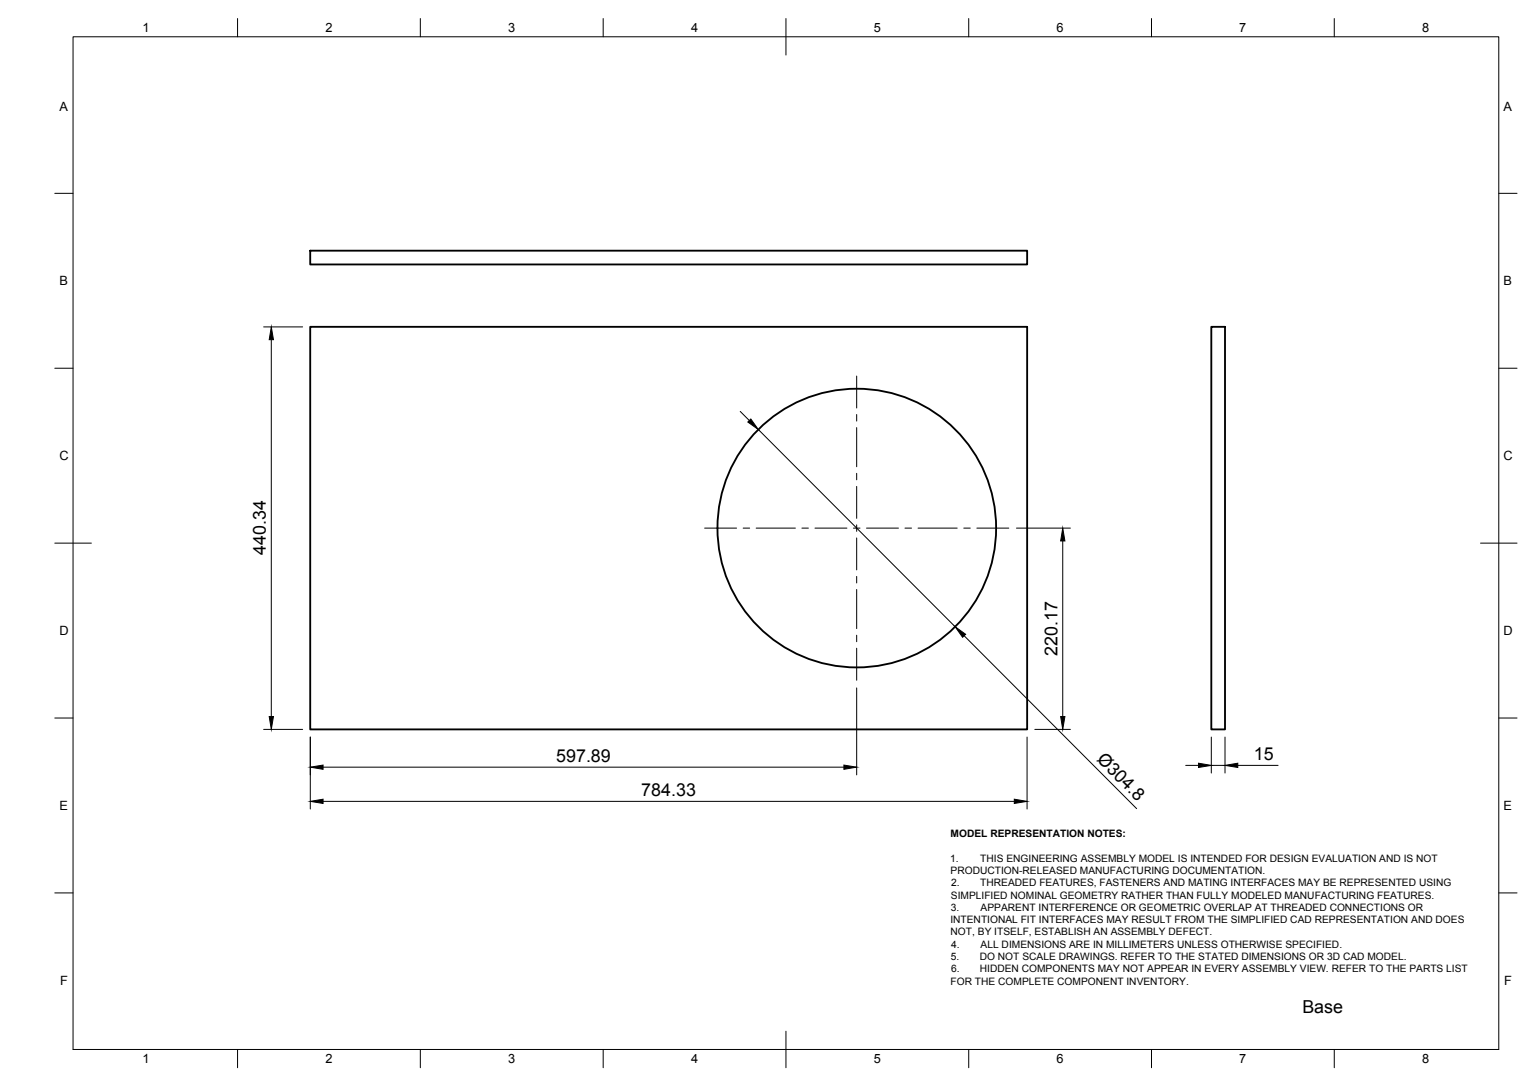
ISO-10303-21;
HEADER;
/* Generated by software containing ST-Developer
 * from STEP Tools, Inc. (www.steptools.com) 
 */

FILE_DESCRIPTION(
/* description */ (''),
/* implementation_level */ '2;1');

FILE_NAME(
/* name */ 'Base.step',
/* time_stamp */ '2026-10-05T19:45:59-07:00',
/* author */ (''),
/* organization */ (''),
/* preprocessor_version */ 'ST-DEVELOPER v20.2',
/* originating_system */ 'Autodesk Translation Framework v15.15.0.0',
/* authorisation */ '');

FILE_SCHEMA (('AUTOMOTIVE_DESIGN { 1 0 10303 214 3 1 1 }'));
ENDSEC;

DATA;
#10=MECHANICAL_DESIGN_GEOMETRIC_PRESENTATION_REPRESENTATION('',(#93),#2462);
#59=FACE_BOUND('',#275,.T.);
#60=FACE_BOUND('',#277,.T.);
#75=SHAPE_REPRESENTATION_RELATIONSHIP('SRR','None',#2501,#84);
#84=ADVANCED_BREP_SHAPE_REPRESENTATION('',(#102),#2456);
#93=STYLED_ITEM('',(#2553),#102);
#102=MANIFOLD_SOLID_BREP('Body1',#1330);
#122=PLANE('',#1482);
#123=PLANE('',#1483);
#124=PLANE('',#1484);
#125=PLANE('',#1485);
#126=PLANE('',#1486);
#127=PLANE('',#1487);
#187=FACE_OUTER_BOUND('',#269,.T.);
#188=FACE_OUTER_BOUND('',#270,.T.);
#189=FACE_OUTER_BOUND('',#271,.T.);
#190=FACE_OUTER_BOUND('',#272,.T.);
#191=FACE_OUTER_BOUND('',#273,.T.);
#192=FACE_OUTER_BOUND('',#274,.T.);
#193=FACE_OUTER_BOUND('',#276,.T.);
#269=EDGE_LOOP('',(#978,#979,#980,#981));
#270=EDGE_LOOP('',(#982,#983,#984,#985));
#271=EDGE_LOOP('',(#986,#987,#988,#989));
#272=EDGE_LOOP('',(#990,#991,#992,#993));
#273=EDGE_LOOP('',(#994,#995,#996,#997));
#274=EDGE_LOOP('',(#998,#999,#1000,#1001));
#275=EDGE_LOOP('',(#1002));
#276=EDGE_LOOP('',(#1003,#1004,#1005,#1006));
#277=EDGE_LOOP('',(#1007));
#366=LINE('',#2085,#485);
#367=LINE('',#2090,#486);
#368=LINE('',#2092,#487);
#369=LINE('',#2094,#488);
#370=LINE('',#2095,#489);
#371=LINE('',#2098,#490);
#372=LINE('',#2100,#491);
#373=LINE('',#2101,#492);
#374=LINE('',#2104,#493);
#375=LINE('',#2106,#494);
#376=LINE('',#2107,#495);
#377=LINE('',#2109,#496);
#378=LINE('',#2110,#497);
#485=VECTOR('',#1695,152.4);
#486=VECTOR('',#1700,10.);
#487=VECTOR('',#1701,10.);
#488=VECTOR('',#1702,10.);
#489=VECTOR('',#1703,10.);
#490=VECTOR('',#1706,10.);
#491=VECTOR('',#1707,10.);
#492=VECTOR('',#1708,10.);
#493=VECTOR('',#1711,10.);
#494=VECTOR('',#1712,10.);
#495=VECTOR('',#1713,10.);
#496=VECTOR('',#1716,10.);
#497=VECTOR('',#1717,10.);
#594=CIRCLE('',#1480,152.4);
#595=CIRCLE('',#1481,152.4);
#649=VERTEX_POINT('',#2082);
#650=VERTEX_POINT('',#2084);
#651=VERTEX_POINT('',#2088);
#652=VERTEX_POINT('',#2089);
#653=VERTEX_POINT('',#2091);
#654=VERTEX_POINT('',#2093);
#655=VERTEX_POINT('',#2097);
#656=VERTEX_POINT('',#2099);
#657=VERTEX_POINT('',#2103);
#658=VERTEX_POINT('',#2105);
#770=EDGE_CURVE('',#649,#649,#594,.T.);
#771=EDGE_CURVE('',#649,#650,#366,.T.);
#772=EDGE_CURVE('',#650,#650,#595,.T.);
#773=EDGE_CURVE('',#651,#652,#367,.T.);
#774=EDGE_CURVE('',#652,#653,#368,.T.);
#775=EDGE_CURVE('',#654,#653,#369,.T.);
#776=EDGE_CURVE('',#651,#654,#370,.T.);
#777=EDGE_CURVE('',#655,#651,#371,.T.);
#778=EDGE_CURVE('',#656,#654,#372,.T.);
#779=EDGE_CURVE('',#655,#656,#373,.T.);
#780=EDGE_CURVE('',#657,#655,#374,.T.);
#781=EDGE_CURVE('',#658,#656,#375,.T.);
#782=EDGE_CURVE('',#657,#658,#376,.T.);
#783=EDGE_CURVE('',#652,#657,#377,.T.);
#784=EDGE_CURVE('',#653,#658,#378,.T.);
#978=ORIENTED_EDGE('',*,*,#770,.T.);
#979=ORIENTED_EDGE('',*,*,#771,.T.);
#980=ORIENTED_EDGE('',*,*,#772,.F.);
#981=ORIENTED_EDGE('',*,*,#771,.F.);
#982=ORIENTED_EDGE('',*,*,#773,.T.);
#983=ORIENTED_EDGE('',*,*,#774,.T.);
#984=ORIENTED_EDGE('',*,*,#775,.F.);
#985=ORIENTED_EDGE('',*,*,#776,.F.);
#986=ORIENTED_EDGE('',*,*,#777,.T.);
#987=ORIENTED_EDGE('',*,*,#776,.T.);
#988=ORIENTED_EDGE('',*,*,#778,.F.);
#989=ORIENTED_EDGE('',*,*,#779,.F.);
#990=ORIENTED_EDGE('',*,*,#780,.T.);
#991=ORIENTED_EDGE('',*,*,#779,.T.);
#992=ORIENTED_EDGE('',*,*,#781,.F.);
#993=ORIENTED_EDGE('',*,*,#782,.F.);
#994=ORIENTED_EDGE('',*,*,#783,.T.);
#995=ORIENTED_EDGE('',*,*,#782,.T.);
#996=ORIENTED_EDGE('',*,*,#784,.F.);
#997=ORIENTED_EDGE('',*,*,#774,.F.);
#998=ORIENTED_EDGE('',*,*,#784,.T.);
#999=ORIENTED_EDGE('',*,*,#781,.T.);
#1000=ORIENTED_EDGE('',*,*,#778,.T.);
#1001=ORIENTED_EDGE('',*,*,#775,.T.);
#1002=ORIENTED_EDGE('',*,*,#772,.T.);
#1003=ORIENTED_EDGE('',*,*,#783,.F.);
#1004=ORIENTED_EDGE('',*,*,#773,.F.);
#1005=ORIENTED_EDGE('',*,*,#777,.F.);
#1006=ORIENTED_EDGE('',*,*,#780,.F.);
#1007=ORIENTED_EDGE('',*,*,#770,.F.);
#1234=CYLINDRICAL_SURFACE('',#1479,152.4);
#1269=ADVANCED_FACE('',(#187),#1234,.F.);
#1270=ADVANCED_FACE('',(#188),#122,.T.);
#1271=ADVANCED_FACE('',(#189),#123,.T.);
#1272=ADVANCED_FACE('',(#190),#124,.T.);
#1273=ADVANCED_FACE('',(#191),#125,.T.);
#1274=ADVANCED_FACE('',(#192,#59),#126,.T.);
#1275=ADVANCED_FACE('',(#193,#60),#127,.F.);
#1330=CLOSED_SHELL('',(#1269,#1270,#1271,#1272,#1273,#1274,#1275));
#1478=AXIS2_PLACEMENT_3D('',#2080,#1689,#1690);
#1479=AXIS2_PLACEMENT_3D('',#2081,#1691,#1692);
#1480=AXIS2_PLACEMENT_3D('',#2083,#1693,#1694);
#1481=AXIS2_PLACEMENT_3D('',#2086,#1696,#1697);
#1482=AXIS2_PLACEMENT_3D('',#2087,#1698,#1699);
#1483=AXIS2_PLACEMENT_3D('',#2096,#1704,#1705);
#1484=AXIS2_PLACEMENT_3D('',#2102,#1709,#1710);
#1485=AXIS2_PLACEMENT_3D('',#2108,#1714,#1715);
#1486=AXIS2_PLACEMENT_3D('',#2111,#1718,#1719);
#1487=AXIS2_PLACEMENT_3D('',#2112,#1720,#1721);
#1689=DIRECTION('axis',(0.,0.,1.));
#1690=DIRECTION('refdir',(1.,0.,0.));
#1691=DIRECTION('center_axis',(0.,0.,-1.));
#1692=DIRECTION('ref_axis',(-1.,0.,0.));
#1693=DIRECTION('center_axis',(0.,0.,1.));
#1694=DIRECTION('ref_axis',(-1.,0.,0.));
#1695=DIRECTION('',(0.,0.,-1.));
#1696=DIRECTION('center_axis',(0.,0.,1.));
#1697=DIRECTION('ref_axis',(-1.,0.,0.));
#1698=DIRECTION('center_axis',(0.,-1.,0.));
#1699=DIRECTION('ref_axis',(-1.,0.,0.));
#1700=DIRECTION('',(-1.,0.,0.));
#1701=DIRECTION('',(0.,0.,-1.));
#1702=DIRECTION('',(-1.,0.,0.));
#1703=DIRECTION('',(0.,0.,-1.));
#1704=DIRECTION('center_axis',(1.,0.,0.));
#1705=DIRECTION('ref_axis',(0.,-1.,0.));
#1706=DIRECTION('',(0.,-1.,0.));
#1707=DIRECTION('',(0.,-1.,0.));
#1708=DIRECTION('',(0.,0.,-1.));
#1709=DIRECTION('center_axis',(0.,1.,0.));
#1710=DIRECTION('ref_axis',(1.,0.,0.));
#1711=DIRECTION('',(1.,0.,0.));
#1712=DIRECTION('',(1.,0.,0.));
#1713=DIRECTION('',(0.,0.,-1.));
#1714=DIRECTION('center_axis',(-1.,0.,0.));
#1715=DIRECTION('ref_axis',(0.,1.,0.));
#1716=DIRECTION('',(0.,1.,0.));
#1717=DIRECTION('',(0.,1.,0.));
#1718=DIRECTION('center_axis',(0.,0.,-1.));
#1719=DIRECTION('ref_axis',(-1.,0.,0.));
#1720=DIRECTION('center_axis',(0.,0.,-1.));
#1721=DIRECTION('ref_axis',(-1.,0.,0.));
#2080=CARTESIAN_POINT('',(0.,0.,0.));
#2081=CARTESIAN_POINT('Origin',(-205.724822686805,0.,-20.));
#2082=CARTESIAN_POINT('',(-53.3248226868051,-1.86636172190057E-14,-20.));
#2083=CARTESIAN_POINT('Origin',(-205.724822686805,0.,-20.));
#2084=CARTESIAN_POINT('',(-53.3248226868051,-1.86636172190057E-14,-35.));
#2085=CARTESIAN_POINT('',(-53.324822686805,-1.86636172190057E-14,-20.));
#2086=CARTESIAN_POINT('Origin',(-205.724822686805,0.,-35.));
#2087=CARTESIAN_POINT('Origin',(392.165319346077,-220.171232331321,-20.));
#2088=CARTESIAN_POINT('',(392.165319346077,-220.171232331321,-20.));
#2089=CARTESIAN_POINT('',(-392.165319346077,-220.171232331321,-20.));
#2090=CARTESIAN_POINT('',(392.165319346077,-220.171232331321,-20.));
#2091=CARTESIAN_POINT('',(-392.165319346077,-220.171232331321,-35.));
#2092=CARTESIAN_POINT('',(-392.165319346077,-220.171232331321,-20.));
#2093=CARTESIAN_POINT('',(392.165319346077,-220.171232331321,-35.));
#2094=CARTESIAN_POINT('',(392.165319346077,-220.171232331321,-35.));
#2095=CARTESIAN_POINT('',(392.165319346077,-220.171232331321,-20.));
#2096=CARTESIAN_POINT('Origin',(392.165319346077,220.171232331321,-20.));
#2097=CARTESIAN_POINT('',(392.165319346077,220.171232331321,-20.));
#2098=CARTESIAN_POINT('',(392.165319346077,220.171232331321,-20.));
#2099=CARTESIAN_POINT('',(392.165319346077,220.171232331321,-35.));
#2100=CARTESIAN_POINT('',(392.165319346077,220.171232331321,-35.));
#2101=CARTESIAN_POINT('',(392.165319346077,220.171232331321,-20.));
#2102=CARTESIAN_POINT('Origin',(-392.165319346077,220.171232331321,-20.));
#2103=CARTESIAN_POINT('',(-392.165319346077,220.171232331321,-20.));
#2104=CARTESIAN_POINT('',(-392.165319346077,220.171232331321,-20.));
#2105=CARTESIAN_POINT('',(-392.165319346077,220.171232331321,-35.));
#2106=CARTESIAN_POINT('',(-392.165319346077,220.171232331321,-35.));
#2107=CARTESIAN_POINT('',(-392.165319346077,220.171232331321,-20.));
#2108=CARTESIAN_POINT('Origin',(-392.165319346077,-220.171232331321,-20.));
#2109=CARTESIAN_POINT('',(-392.165319346077,-220.171232331321,-20.));
#2110=CARTESIAN_POINT('',(-392.165319346077,-220.171232331321,-35.));
#2111=CARTESIAN_POINT('Origin',(0.,0.,-35.));
#2112=CARTESIAN_POINT('Origin',(0.,0.,-20.));
#2445=UNCERTAINTY_MEASURE_WITH_UNIT(LENGTH_MEASURE(0.01),#2463,
'DISTANCE_ACCURACY_VALUE',
'Maximum model space distance between geometric entities at asserted c
onnectivities');
#2451=UNCERTAINTY_MEASURE_WITH_UNIT(LENGTH_MEASURE(0.01),#2463,
'DISTANCE_ACCURACY_VALUE',
'Maximum model space distance between geometric entities at asserted c
onnectivities');
#2456=(
GEOMETRIC_REPRESENTATION_CONTEXT(3)
GLOBAL_UNCERTAINTY_ASSIGNED_CONTEXT((#2445))
GLOBAL_UNIT_ASSIGNED_CONTEXT((#2463,#2465,#2466))
REPRESENTATION_CONTEXT('','3D')
);
#2462=(
GEOMETRIC_REPRESENTATION_CONTEXT(3)
GLOBAL_UNCERTAINTY_ASSIGNED_CONTEXT((#2451))
GLOBAL_UNIT_ASSIGNED_CONTEXT((#2463,#2465,#2466))
REPRESENTATION_CONTEXT('','3D')
);
#2463=(
LENGTH_UNIT()
NAMED_UNIT(*)
SI_UNIT(.MILLI.,.METRE.)
);
#2465=(
NAMED_UNIT(*)
PLANE_ANGLE_UNIT()
SI_UNIT($,.RADIAN.)
);
#2466=(
NAMED_UNIT(*)
SI_UNIT($,.STERADIAN.)
SOLID_ANGLE_UNIT()
);
#2471=SHAPE_DEFINITION_REPRESENTATION(#2481,#2501);
#2481=PRODUCT_DEFINITION_SHAPE('',$,#2512);
#2501=SHAPE_REPRESENTATION('',(#1478),#2456);
#2507=PRODUCT_DEFINITION_CONTEXT('part definition',#2539,'design');
#2512=PRODUCT_DEFINITION('base','Base',#2522,#2507);
#2522=PRODUCT_DEFINITION_FORMATION('',$,#2545);
#2539=APPLICATION_CONTEXT(
'Core Data for Automotive Mechanical Design Process');
#2540=PRODUCT_CONTEXT('part definition',#2539,'mechanical');
#2545=PRODUCT('base','Base',$,(#2540));
#2553=PRESENTATION_STYLE_ASSIGNMENT((#2556));
#2556=SURFACE_STYLE_USAGE(.BOTH.,#2559);
#2559=SURFACE_SIDE_STYLE('',(#2562));
#2562=SURFACE_STYLE_FILL_AREA(#2565);
#2565=FILL_AREA_STYLE('Opaque(179,179,179)',(#2568));
#2568=FILL_AREA_STYLE_COLOUR('Opaque(179,179,179)',#2571);
#2571=COLOUR_RGB('Opaque(179,179,179)', 0.31764706, 0.68627451, 0.89019608);
ENDSEC;
END-ISO-10303-21;
